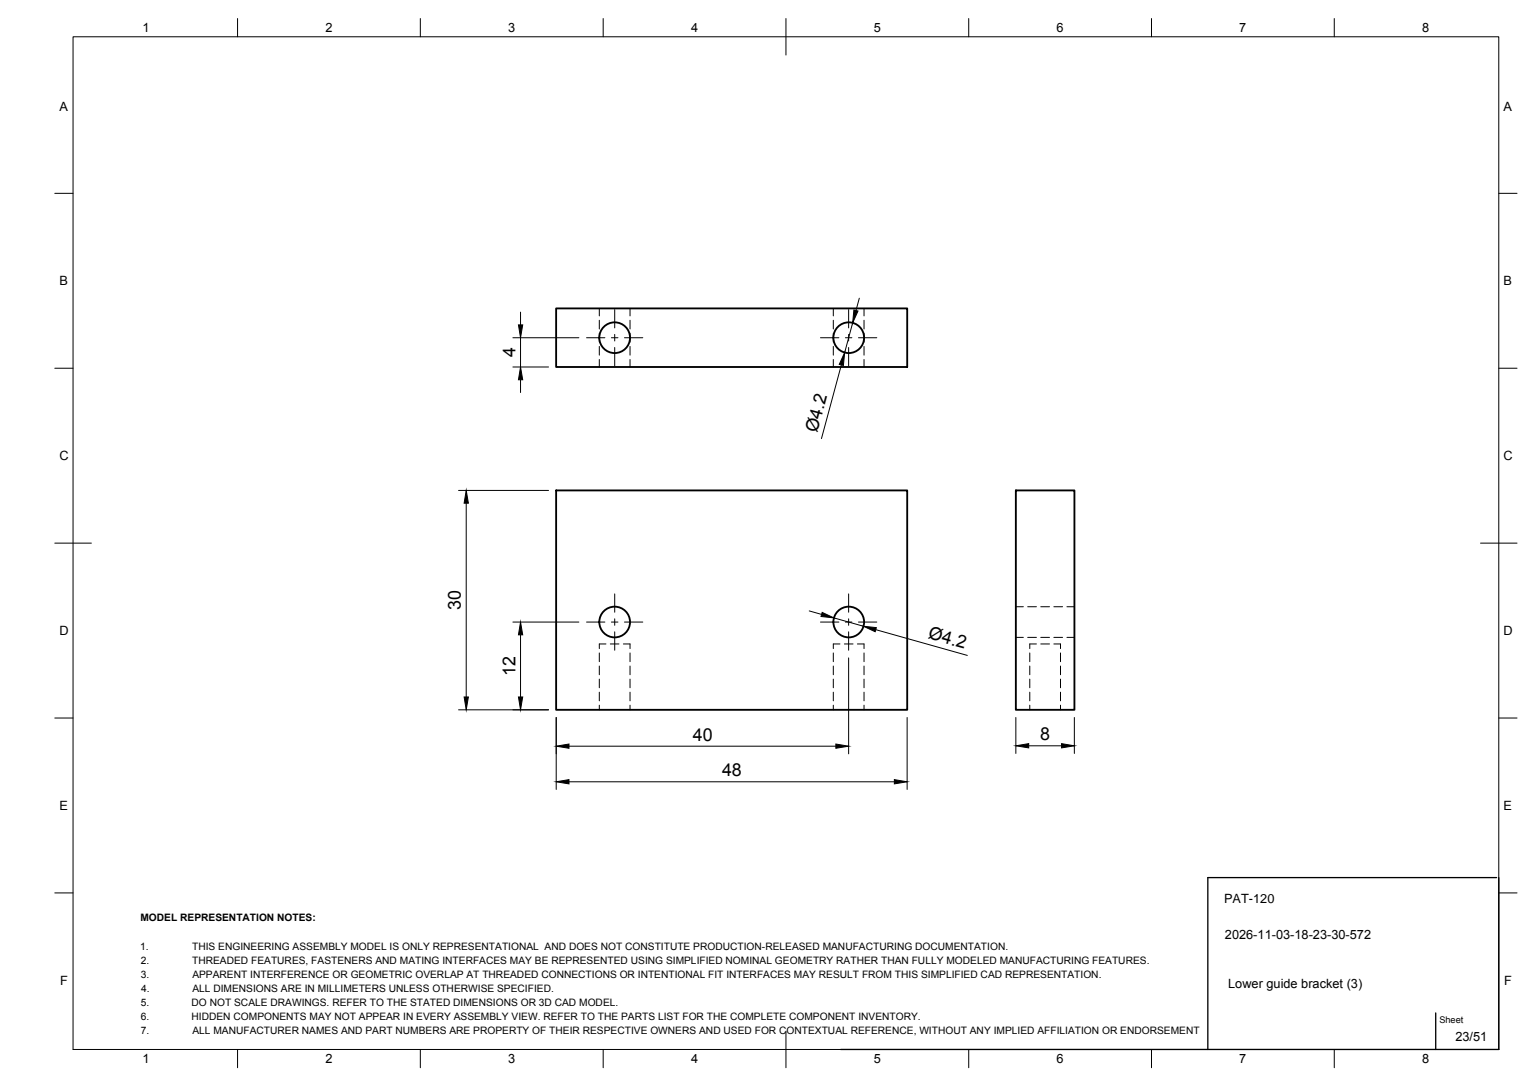
ISO-10303-21;
HEADER;
/* Generated by software containing ST-Developer
 * from STEP Tools, Inc. (www.steptools.com) 
 */

FILE_DESCRIPTION(
/* description */ ('Vibration shaker table dummy'),
/* implementation_level */ '2;1');

FILE_NAME(
/* name */ 'Lower guide bracket (3).step',
/* time_stamp */ '2026-10-27T10:55:14-07:00',
/* author */ (''),
/* organization */ (''),
/* preprocessor_version */ 'ST-DEVELOPER v20.2',
/* originating_system */ 'Autodesk Translation Framework v15.17.0.0',
/* authorisation */ '');

FILE_SCHEMA (('AUTOMOTIVE_DESIGN { 1 0 10303 214 3 1 1 }'));
ENDSEC;

DATA;
#10=MECHANICAL_DESIGN_GEOMETRIC_PRESENTATION_REPRESENTATION('',(#704),#22394);
#612=SHAPE_REPRESENTATION_RELATIONSHIP('SRR','None',#22658,#658);
#658=ADVANCED_BREP_SHAPE_REPRESENTATION('',(#750),#22364);
#704=STYLED_ITEM('',(#22940),#750);
#750=MANIFOLD_SOLID_BREP('Body1',#9222);
#905=FACE_BOUND('',#2167,.T.);
#906=FACE_BOUND('',#2168,.T.);
#907=FACE_BOUND('',#2171,.T.);
#908=FACE_BOUND('',#2172,.T.);
#909=FACE_BOUND('',#2176,.T.);
#910=FACE_BOUND('',#2177,.T.);
#1170=PLANE('',#10146);
#1171=PLANE('',#10150);
#1172=PLANE('',#10157);
#1173=PLANE('',#10158);
#1174=PLANE('',#10159);
#1175=PLANE('',#10160);
#1176=PLANE('',#10161);
#1177=PLANE('',#10162);
#1532=FACE_OUTER_BOUND('',#2160,.T.);
#1533=FACE_OUTER_BOUND('',#2161,.T.);
#1534=FACE_OUTER_BOUND('',#2162,.T.);
#1535=FACE_OUTER_BOUND('',#2163,.T.);
#1536=FACE_OUTER_BOUND('',#2164,.T.);
#1537=FACE_OUTER_BOUND('',#2165,.T.);
#1538=FACE_OUTER_BOUND('',#2166,.T.);
#1539=FACE_OUTER_BOUND('',#2169,.T.);
#1540=FACE_OUTER_BOUND('',#2170,.T.);
#1541=FACE_OUTER_BOUND('',#2173,.T.);
#1542=FACE_OUTER_BOUND('',#2174,.T.);
#1543=FACE_OUTER_BOUND('',#2175,.T.);
#2160=EDGE_LOOP('',(#7128,#7129,#7130,#7131));
#2161=EDGE_LOOP('',(#7132));
#2162=EDGE_LOOP('',(#7133,#7134,#7135,#7136));
#2163=EDGE_LOOP('',(#7137));
#2164=EDGE_LOOP('',(#7138,#7139,#7140,#7141));
#2165=EDGE_LOOP('',(#7142,#7143,#7144,#7145));
#2166=EDGE_LOOP('',(#7146,#7147,#7148,#7149));
#2167=EDGE_LOOP('',(#7150));
#2168=EDGE_LOOP('',(#7151));
#2169=EDGE_LOOP('',(#7152,#7153,#7154,#7155));
#2170=EDGE_LOOP('',(#7156,#7157,#7158,#7159));
#2171=EDGE_LOOP('',(#7160));
#2172=EDGE_LOOP('',(#7161));
#2173=EDGE_LOOP('',(#7162,#7163,#7164,#7165));
#2174=EDGE_LOOP('',(#7166,#7167,#7168,#7169));
#2175=EDGE_LOOP('',(#7170,#7171,#7172,#7173));
#2176=EDGE_LOOP('',(#7174));
#2177=EDGE_LOOP('',(#7175));
#2886=LINE('',#19283,#3505);
#2887=LINE('',#19290,#3506);
#2888=LINE('',#19297,#3507);
#2889=LINE('',#19303,#3508);
#2890=LINE('',#19308,#3509);
#2891=LINE('',#19310,#3510);
#2892=LINE('',#19312,#3511);
#2893=LINE('',#19313,#3512);
#2894=LINE('',#19316,#3513);
#2895=LINE('',#19318,#3514);
#2896=LINE('',#19319,#3515);
#2897=LINE('',#19322,#3516);
#2898=LINE('',#19324,#3517);
#2899=LINE('',#19325,#3518);
#2900=LINE('',#19327,#3519);
#2901=LINE('',#19328,#3520);
#3505=VECTOR('',#11984,0.21);
#3506=VECTOR('',#11993,0.21);
#3507=VECTOR('',#12002,0.21);
#3508=VECTOR('',#12009,0.21);
#3509=VECTOR('',#12014,1.);
#3510=VECTOR('',#12015,1.);
#3511=VECTOR('',#12016,1.);
#3512=VECTOR('',#12017,1.);
#3513=VECTOR('',#12020,1.);
#3514=VECTOR('',#12021,1.);
#3515=VECTOR('',#12022,1.);
#3516=VECTOR('',#12025,1.);
#3517=VECTOR('',#12026,1.);
#3518=VECTOR('',#12027,1.);
#3519=VECTOR('',#12030,1.);
#3520=VECTOR('',#12031,1.);
#4034=CIRCLE('',#10144,0.21);
#4035=CIRCLE('',#10145,0.21);
#4036=CIRCLE('',#10148,0.21);
#4037=CIRCLE('',#10149,0.21);
#4038=CIRCLE('',#10152,0.21);
#4039=CIRCLE('',#10153,0.21);
#4040=CIRCLE('',#10155,0.21);
#4041=CIRCLE('',#10156,0.21);
#4661=VERTEX_POINT('',#19280);
#4662=VERTEX_POINT('',#19282);
#4663=VERTEX_POINT('',#19287);
#4664=VERTEX_POINT('',#19289);
#4665=VERTEX_POINT('',#19294);
#4666=VERTEX_POINT('',#19296);
#4667=VERTEX_POINT('',#19300);
#4668=VERTEX_POINT('',#19302);
#4669=VERTEX_POINT('',#19306);
#4670=VERTEX_POINT('',#19307);
#4671=VERTEX_POINT('',#19309);
#4672=VERTEX_POINT('',#19311);
#4673=VERTEX_POINT('',#19315);
#4674=VERTEX_POINT('',#19317);
#4675=VERTEX_POINT('',#19321);
#4676=VERTEX_POINT('',#19323);
#5557=EDGE_CURVE('',#4661,#4661,#4034,.T.);
#5558=EDGE_CURVE('',#4661,#4662,#2886,.T.);
#5559=EDGE_CURVE('',#4662,#4662,#4035,.T.);
#5560=EDGE_CURVE('',#4663,#4663,#4036,.T.);
#5561=EDGE_CURVE('',#4663,#4664,#2887,.T.);
#5562=EDGE_CURVE('',#4664,#4664,#4037,.T.);
#5563=EDGE_CURVE('',#4665,#4665,#4038,.T.);
#5564=EDGE_CURVE('',#4665,#4666,#2888,.T.);
#5565=EDGE_CURVE('',#4666,#4666,#4039,.T.);
#5566=EDGE_CURVE('',#4667,#4667,#4040,.T.);
#5567=EDGE_CURVE('',#4667,#4668,#2889,.T.);
#5568=EDGE_CURVE('',#4668,#4668,#4041,.T.);
#5569=EDGE_CURVE('',#4669,#4670,#2890,.T.);
#5570=EDGE_CURVE('',#4670,#4671,#2891,.T.);
#5571=EDGE_CURVE('',#4672,#4671,#2892,.T.);
#5572=EDGE_CURVE('',#4669,#4672,#2893,.T.);
#5573=EDGE_CURVE('',#4673,#4669,#2894,.T.);
#5574=EDGE_CURVE('',#4674,#4672,#2895,.T.);
#5575=EDGE_CURVE('',#4673,#4674,#2896,.T.);
#5576=EDGE_CURVE('',#4675,#4673,#2897,.T.);
#5577=EDGE_CURVE('',#4676,#4674,#2898,.T.);
#5578=EDGE_CURVE('',#4675,#4676,#2899,.T.);
#5579=EDGE_CURVE('',#4670,#4675,#2900,.T.);
#5580=EDGE_CURVE('',#4671,#4676,#2901,.T.);
#7128=ORIENTED_EDGE('',*,*,#5557,.F.);
#7129=ORIENTED_EDGE('',*,*,#5558,.T.);
#7130=ORIENTED_EDGE('',*,*,#5559,.T.);
#7131=ORIENTED_EDGE('',*,*,#5558,.F.);
#7132=ORIENTED_EDGE('',*,*,#5559,.F.);
#7133=ORIENTED_EDGE('',*,*,#5560,.F.);
#7134=ORIENTED_EDGE('',*,*,#5561,.T.);
#7135=ORIENTED_EDGE('',*,*,#5562,.T.);
#7136=ORIENTED_EDGE('',*,*,#5561,.F.);
#7137=ORIENTED_EDGE('',*,*,#5562,.F.);
#7138=ORIENTED_EDGE('',*,*,#5563,.F.);
#7139=ORIENTED_EDGE('',*,*,#5564,.T.);
#7140=ORIENTED_EDGE('',*,*,#5565,.F.);
#7141=ORIENTED_EDGE('',*,*,#5564,.F.);
#7142=ORIENTED_EDGE('',*,*,#5566,.F.);
#7143=ORIENTED_EDGE('',*,*,#5567,.T.);
#7144=ORIENTED_EDGE('',*,*,#5568,.F.);
#7145=ORIENTED_EDGE('',*,*,#5567,.F.);
#7146=ORIENTED_EDGE('',*,*,#5569,.T.);
#7147=ORIENTED_EDGE('',*,*,#5570,.T.);
#7148=ORIENTED_EDGE('',*,*,#5571,.F.);
#7149=ORIENTED_EDGE('',*,*,#5572,.F.);
#7150=ORIENTED_EDGE('',*,*,#5565,.T.);
#7151=ORIENTED_EDGE('',*,*,#5568,.T.);
#7152=ORIENTED_EDGE('',*,*,#5573,.T.);
#7153=ORIENTED_EDGE('',*,*,#5572,.T.);
#7154=ORIENTED_EDGE('',*,*,#5574,.F.);
#7155=ORIENTED_EDGE('',*,*,#5575,.F.);
#7156=ORIENTED_EDGE('',*,*,#5576,.T.);
#7157=ORIENTED_EDGE('',*,*,#5575,.T.);
#7158=ORIENTED_EDGE('',*,*,#5577,.F.);
#7159=ORIENTED_EDGE('',*,*,#5578,.F.);
#7160=ORIENTED_EDGE('',*,*,#5563,.T.);
#7161=ORIENTED_EDGE('',*,*,#5566,.T.);
#7162=ORIENTED_EDGE('',*,*,#5579,.T.);
#7163=ORIENTED_EDGE('',*,*,#5578,.T.);
#7164=ORIENTED_EDGE('',*,*,#5580,.F.);
#7165=ORIENTED_EDGE('',*,*,#5570,.F.);
#7166=ORIENTED_EDGE('',*,*,#5580,.T.);
#7167=ORIENTED_EDGE('',*,*,#5577,.T.);
#7168=ORIENTED_EDGE('',*,*,#5574,.T.);
#7169=ORIENTED_EDGE('',*,*,#5571,.T.);
#7170=ORIENTED_EDGE('',*,*,#5579,.F.);
#7171=ORIENTED_EDGE('',*,*,#5569,.F.);
#7172=ORIENTED_EDGE('',*,*,#5573,.F.);
#7173=ORIENTED_EDGE('',*,*,#5576,.F.);
#7174=ORIENTED_EDGE('',*,*,#5557,.T.);
#7175=ORIENTED_EDGE('',*,*,#5560,.T.);
#8584=CYLINDRICAL_SURFACE('',#10143,0.21);
#8585=CYLINDRICAL_SURFACE('',#10147,0.21);
#8586=CYLINDRICAL_SURFACE('',#10151,0.21);
#8587=CYLINDRICAL_SURFACE('',#10154,0.21);
#8897=ADVANCED_FACE('',(#1532),#8584,.F.);
#8898=ADVANCED_FACE('',(#1533),#1170,.F.);
#8899=ADVANCED_FACE('',(#1534),#8585,.F.);
#8900=ADVANCED_FACE('',(#1535),#1171,.F.);
#8901=ADVANCED_FACE('',(#1536),#8586,.F.);
#8902=ADVANCED_FACE('',(#1537),#8587,.F.);
#8903=ADVANCED_FACE('',(#1538,#905,#906),#1172,.T.);
#8904=ADVANCED_FACE('',(#1539),#1173,.T.);
#8905=ADVANCED_FACE('',(#1540,#907,#908),#1174,.T.);
#8906=ADVANCED_FACE('',(#1541),#1175,.T.);
#8907=ADVANCED_FACE('',(#1542),#1176,.T.);
#8908=ADVANCED_FACE('',(#1543,#909,#910),#1177,.F.);
#9222=CLOSED_SHELL('',(#8897,#8898,#8899,#8900,#8901,#8902,#8903,#8904,
#8905,#8906,#8907,#8908));
#10142=AXIS2_PLACEMENT_3D('',#19278,#11978,#11979);
#10143=AXIS2_PLACEMENT_3D('',#19279,#11980,#11981);
#10144=AXIS2_PLACEMENT_3D('',#19281,#11982,#11983);
#10145=AXIS2_PLACEMENT_3D('',#19284,#11985,#11986);
#10146=AXIS2_PLACEMENT_3D('',#19285,#11987,#11988);
#10147=AXIS2_PLACEMENT_3D('',#19286,#11989,#11990);
#10148=AXIS2_PLACEMENT_3D('',#19288,#11991,#11992);
#10149=AXIS2_PLACEMENT_3D('',#19291,#11994,#11995);
#10150=AXIS2_PLACEMENT_3D('',#19292,#11996,#11997);
#10151=AXIS2_PLACEMENT_3D('',#19293,#11998,#11999);
#10152=AXIS2_PLACEMENT_3D('',#19295,#12000,#12001);
#10153=AXIS2_PLACEMENT_3D('',#19298,#12003,#12004);
#10154=AXIS2_PLACEMENT_3D('',#19299,#12005,#12006);
#10155=AXIS2_PLACEMENT_3D('',#19301,#12007,#12008);
#10156=AXIS2_PLACEMENT_3D('',#19304,#12010,#12011);
#10157=AXIS2_PLACEMENT_3D('',#19305,#12012,#12013);
#10158=AXIS2_PLACEMENT_3D('',#19314,#12018,#12019);
#10159=AXIS2_PLACEMENT_3D('',#19320,#12023,#12024);
#10160=AXIS2_PLACEMENT_3D('',#19326,#12028,#12029);
#10161=AXIS2_PLACEMENT_3D('',#19329,#12032,#12033);
#10162=AXIS2_PLACEMENT_3D('',#19330,#12034,#12035);
#11978=DIRECTION('axis',(0.,0.,1.));
#11979=DIRECTION('refdir',(1.,0.,0.));
#11980=DIRECTION('center_axis',(0.,0.,1.));
#11981=DIRECTION('ref_axis',(1.,0.,0.));
#11982=DIRECTION('center_axis',(0.,0.,1.));
#11983=DIRECTION('ref_axis',(1.,0.,0.));
#11984=DIRECTION('',(0.,0.,1.));
#11985=DIRECTION('center_axis',(0.,0.,1.));
#11986=DIRECTION('ref_axis',(1.,0.,0.));
#11987=DIRECTION('center_axis',(0.,0.,1.));
#11988=DIRECTION('ref_axis',(1.,0.,0.));
#11989=DIRECTION('center_axis',(0.,0.,1.));
#11990=DIRECTION('ref_axis',(1.,0.,0.));
#11991=DIRECTION('center_axis',(0.,0.,1.));
#11992=DIRECTION('ref_axis',(1.,0.,0.));
#11993=DIRECTION('',(0.,0.,1.));
#11994=DIRECTION('center_axis',(0.,0.,1.));
#11995=DIRECTION('ref_axis',(1.,0.,0.));
#11996=DIRECTION('center_axis',(0.,0.,1.));
#11997=DIRECTION('ref_axis',(1.,0.,0.));
#11998=DIRECTION('center_axis',(0.,1.,0.));
#11999=DIRECTION('ref_axis',(1.,0.,0.));
#12000=DIRECTION('center_axis',(0.,1.,0.));
#12001=DIRECTION('ref_axis',(1.,0.,0.));
#12002=DIRECTION('',(0.,1.,0.));
#12003=DIRECTION('center_axis',(0.,-1.,0.));
#12004=DIRECTION('ref_axis',(1.,0.,0.));
#12005=DIRECTION('center_axis',(0.,1.,0.));
#12006=DIRECTION('ref_axis',(1.,0.,0.));
#12007=DIRECTION('center_axis',(0.,1.,0.));
#12008=DIRECTION('ref_axis',(1.,0.,0.));
#12009=DIRECTION('',(0.,1.,0.));
#12010=DIRECTION('center_axis',(0.,-1.,0.));
#12011=DIRECTION('ref_axis',(1.,0.,0.));
#12012=DIRECTION('center_axis',(0.,1.,0.));
#12013=DIRECTION('ref_axis',(-1.,0.,0.));
#12014=DIRECTION('',(-1.,0.,0.));
#12015=DIRECTION('',(0.,0.,1.));
#12016=DIRECTION('',(-1.,0.,0.));
#12017=DIRECTION('',(0.,0.,1.));
#12018=DIRECTION('center_axis',(1.,0.,0.));
#12019=DIRECTION('ref_axis',(0.,1.,0.));
#12020=DIRECTION('',(0.,1.,0.));
#12021=DIRECTION('',(0.,1.,0.));
#12022=DIRECTION('',(0.,0.,1.));
#12023=DIRECTION('center_axis',(0.,-1.,0.));
#12024=DIRECTION('ref_axis',(1.,0.,0.));
#12025=DIRECTION('',(1.,0.,0.));
#12026=DIRECTION('',(1.,0.,0.));
#12027=DIRECTION('',(0.,0.,1.));
#12028=DIRECTION('center_axis',(-1.,0.,0.));
#12029=DIRECTION('ref_axis',(0.,-1.,0.));
#12030=DIRECTION('',(0.,-1.,0.));
#12031=DIRECTION('',(0.,-1.,0.));
#12032=DIRECTION('center_axis',(0.,0.,1.));
#12033=DIRECTION('ref_axis',(1.,0.,0.));
#12034=DIRECTION('center_axis',(0.,0.,1.));
#12035=DIRECTION('ref_axis',(1.,0.,0.));
#19278=CARTESIAN_POINT('',(0.,0.,0.));
#19279=CARTESIAN_POINT('Origin',(4.4,6.7,-0.1));
#19280=CARTESIAN_POINT('',(4.19,6.7,0.));
#19281=CARTESIAN_POINT('Origin',(4.4,6.7,0.));
#19282=CARTESIAN_POINT('',(4.19,6.7,0.9));
#19283=CARTESIAN_POINT('',(4.19,6.7,-0.1));
#19284=CARTESIAN_POINT('Origin',(4.4,6.7,0.9));
#19285=CARTESIAN_POINT('Origin',(4.4,6.7,0.9));
#19286=CARTESIAN_POINT('Origin',(7.6,6.7,-0.1));
#19287=CARTESIAN_POINT('',(7.39,6.7,0.));
#19288=CARTESIAN_POINT('Origin',(7.6,6.7,0.));
#19289=CARTESIAN_POINT('',(7.39,6.7,0.9));
#19290=CARTESIAN_POINT('',(7.39,6.7,-0.1));
#19291=CARTESIAN_POINT('Origin',(7.6,6.7,0.9));
#19292=CARTESIAN_POINT('Origin',(7.6,6.7,0.9));
#19293=CARTESIAN_POINT('Origin',(4.4,6.2,1.2));
#19294=CARTESIAN_POINT('',(4.19,6.3,1.2));
#19295=CARTESIAN_POINT('Origin',(4.4,6.3,1.2));
#19296=CARTESIAN_POINT('',(4.19,7.1,1.2));
#19297=CARTESIAN_POINT('',(4.19,6.2,1.2));
#19298=CARTESIAN_POINT('Origin',(4.4,7.1,1.2));
#19299=CARTESIAN_POINT('Origin',(7.6,6.2,1.2));
#19300=CARTESIAN_POINT('',(7.39,6.3,1.2));
#19301=CARTESIAN_POINT('Origin',(7.6,6.3,1.2));
#19302=CARTESIAN_POINT('',(7.39,7.1,1.2));
#19303=CARTESIAN_POINT('',(7.39,6.2,1.2));
#19304=CARTESIAN_POINT('Origin',(7.6,7.1,1.2));
#19305=CARTESIAN_POINT('Origin',(8.4,7.1,0.));
#19306=CARTESIAN_POINT('',(8.4,7.1,0.));
#19307=CARTESIAN_POINT('',(3.6,7.1,0.));
#19308=CARTESIAN_POINT('',(8.4,7.1,0.));
#19309=CARTESIAN_POINT('',(3.6,7.1,3.));
#19310=CARTESIAN_POINT('',(3.6,7.1,0.));
#19311=CARTESIAN_POINT('',(8.4,7.1,3.));
#19312=CARTESIAN_POINT('',(8.4,7.1,3.));
#19313=CARTESIAN_POINT('',(8.4,7.1,0.));
#19314=CARTESIAN_POINT('Origin',(8.4,6.3,0.));
#19315=CARTESIAN_POINT('',(8.4,6.3,0.));
#19316=CARTESIAN_POINT('',(8.4,6.3,0.));
#19317=CARTESIAN_POINT('',(8.4,6.3,3.));
#19318=CARTESIAN_POINT('',(8.4,6.3,3.));
#19319=CARTESIAN_POINT('',(8.4,6.3,0.));
#19320=CARTESIAN_POINT('Origin',(3.6,6.3,0.));
#19321=CARTESIAN_POINT('',(3.6,6.3,0.));
#19322=CARTESIAN_POINT('',(3.6,6.3,0.));
#19323=CARTESIAN_POINT('',(3.6,6.3,3.));
#19324=CARTESIAN_POINT('',(3.6,6.3,3.));
#19325=CARTESIAN_POINT('',(3.6,6.3,0.));
#19326=CARTESIAN_POINT('Origin',(3.6,7.1,0.));
#19327=CARTESIAN_POINT('',(3.6,7.1,0.));
#19328=CARTESIAN_POINT('',(3.6,7.1,3.));
#19329=CARTESIAN_POINT('Origin',(6.,6.7,3.));
#19330=CARTESIAN_POINT('Origin',(6.,6.7,0.));
#22313=UNCERTAINTY_MEASURE_WITH_UNIT(LENGTH_MEASURE(0.001),#22395,
'DISTANCE_ACCURACY_VALUE',
'Maximum model space distance between geometric entities at asserted c
onnectivities');
#22343=UNCERTAINTY_MEASURE_WITH_UNIT(LENGTH_MEASURE(0.001),#22395,
'DISTANCE_ACCURACY_VALUE',
'Maximum model space distance between geometric entities at asserted c
onnectivities');
#22364=(
GEOMETRIC_REPRESENTATION_CONTEXT(3)
GLOBAL_UNCERTAINTY_ASSIGNED_CONTEXT((#22313))
GLOBAL_UNIT_ASSIGNED_CONTEXT((#22395,#22397,#22398))
REPRESENTATION_CONTEXT('','3D')
);
#22394=(
GEOMETRIC_REPRESENTATION_CONTEXT(3)
GLOBAL_UNCERTAINTY_ASSIGNED_CONTEXT((#22343))
GLOBAL_UNIT_ASSIGNED_CONTEXT((#22395,#22397,#22398))
REPRESENTATION_CONTEXT('','3D')
);
#22395=(
LENGTH_UNIT()
NAMED_UNIT(*)
SI_UNIT(.CENTI.,.METRE.)
);
#22397=(
NAMED_UNIT(*)
PLANE_ANGLE_UNIT()
SI_UNIT($,.RADIAN.)
);
#22398=(
NAMED_UNIT(*)
SI_UNIT($,.STERADIAN.)
SOLID_ANGLE_UNIT()
);
#22419=SHAPE_DEFINITION_REPRESENTATION(#22469,#22658);
#22469=PRODUCT_DEFINITION_SHAPE('',$,#22709);
#22658=SHAPE_REPRESENTATION('',(#10142),#22364);
#22688=PRODUCT_DEFINITION_CONTEXT('part definition',#22840,'design');
#22709=PRODUCT_DEFINITION('Lower guide bracket (3)',
'Lower guide bracket (3)',#22759,#22688);
#22759=PRODUCT_DEFINITION_FORMATION('',$,#22862);
#22840=APPLICATION_CONTEXT(
'Core Data for Automotive Mechanical Design Process');
#22841=PRODUCT_CONTEXT('part definition',#22840,'mechanical');
#22862=PRODUCT('Lower guide bracket (3)','Lower guide bracket (3)',
'Lower guide bracket (3)',(#22841));
#22934=COLOUR_RGB('Dark Blue',0.08,0.2,0.34);
#22935=FILL_AREA_STYLE_COLOUR('',#22934);
#22936=FILL_AREA_STYLE('',(#22935));
#22937=SURFACE_STYLE_FILL_AREA(#22936);
#22938=SURFACE_SIDE_STYLE('',(#22937));
#22939=SURFACE_STYLE_USAGE(.BOTH.,#22938);
#22940=PRESENTATION_STYLE_ASSIGNMENT((#22939));
ENDSEC;
END-ISO-10303-21;
